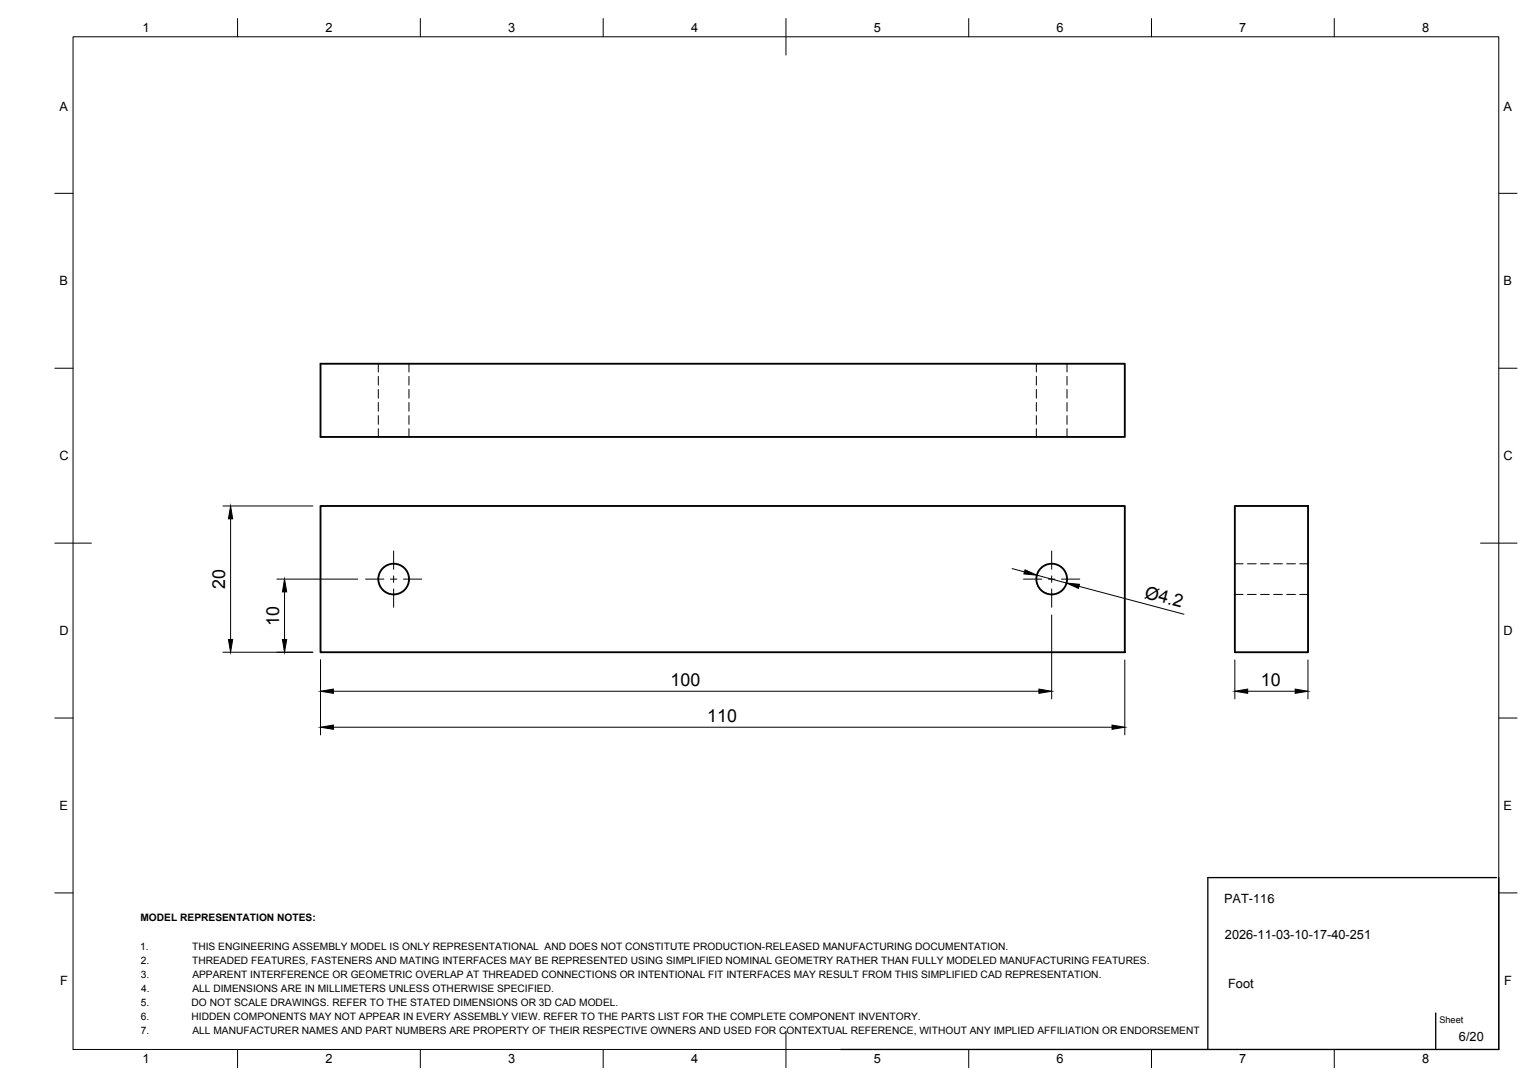
ISO-10303-21;
HEADER;
/* Generated by software containing ST-Developer
 * from STEP Tools, Inc. (www.steptools.com) 
 */

FILE_DESCRIPTION(
/* description */ ('V-block with clamp strap'),
/* implementation_level */ '2;1');

FILE_NAME(
/* name */ 'Foot.step',
/* time_stamp */ '2026-10-27T10:50:53-07:00',
/* author */ (''),
/* organization */ (''),
/* preprocessor_version */ 'ST-DEVELOPER v20.2',
/* originating_system */ 'Autodesk Translation Framework v15.17.0.0',
/* authorisation */ '');

FILE_SCHEMA (('AUTOMOTIVE_DESIGN { 1 0 10303 214 3 1 1 }'));
ENDSEC;

DATA;
#10=MECHANICAL_DESIGN_GEOMETRIC_PRESENTATION_REPRESENTATION('',(#267),#7344);
#225=SHAPE_REPRESENTATION_RELATIONSHIP('SRR','None',#7443,#246);
#246=ADVANCED_BREP_SHAPE_REPRESENTATION('',(#288),#7322);
#267=STYLED_ITEM('',(#7645),#288);
#288=MANIFOLD_SOLID_BREP('Body1',#4149);
#331=FACE_BOUND('',#863,.T.);
#332=FACE_BOUND('',#864,.T.);
#333=FACE_BOUND('',#866,.T.);
#334=FACE_BOUND('',#867,.T.);
#400=CIRCLE('',#4461,0.21);
#401=CIRCLE('',#4462,0.21);
#402=CIRCLE('',#4464,0.21);
#403=CIRCLE('',#4465,0.21);
#517=CYLINDRICAL_SURFACE('',#4460,0.21);
#518=CYLINDRICAL_SURFACE('',#4463,0.21);
#590=FACE_OUTER_BOUND('',#856,.T.);
#591=FACE_OUTER_BOUND('',#857,.T.);
#592=FACE_OUTER_BOUND('',#858,.T.);
#593=FACE_OUTER_BOUND('',#859,.T.);
#594=FACE_OUTER_BOUND('',#860,.T.);
#595=FACE_OUTER_BOUND('',#861,.T.);
#596=FACE_OUTER_BOUND('',#862,.T.);
#597=FACE_OUTER_BOUND('',#865,.T.);
#856=EDGE_LOOP('',(#2840,#2841,#2842,#2843));
#857=EDGE_LOOP('',(#2844,#2845,#2846,#2847));
#858=EDGE_LOOP('',(#2848,#2849,#2850,#2851));
#859=EDGE_LOOP('',(#2852,#2853,#2854,#2855));
#860=EDGE_LOOP('',(#2856,#2857,#2858,#2859));
#861=EDGE_LOOP('',(#2860,#2861,#2862,#2863));
#862=EDGE_LOOP('',(#2864,#2865,#2866,#2867));
#863=EDGE_LOOP('',(#2868));
#864=EDGE_LOOP('',(#2869));
#865=EDGE_LOOP('',(#2870,#2871,#2872,#2873));
#866=EDGE_LOOP('',(#2874));
#867=EDGE_LOOP('',(#2875));
#1161=LINE('',#6242,#1526);
#1162=LINE('',#6248,#1527);
#1163=LINE('',#6253,#1528);
#1164=LINE('',#6255,#1529);
#1165=LINE('',#6257,#1530);
#1166=LINE('',#6258,#1531);
#1167=LINE('',#6261,#1532);
#1168=LINE('',#6263,#1533);
#1169=LINE('',#6264,#1534);
#1170=LINE('',#6267,#1535);
#1171=LINE('',#6269,#1536);
#1172=LINE('',#6270,#1537);
#1173=LINE('',#6272,#1538);
#1174=LINE('',#6273,#1539);
#1526=VECTOR('',#5007,0.21);
#1527=VECTOR('',#5014,0.21);
#1528=VECTOR('',#5019,1.);
#1529=VECTOR('',#5020,1.);
#1530=VECTOR('',#5021,1.);
#1531=VECTOR('',#5022,1.);
#1532=VECTOR('',#5025,1.);
#1533=VECTOR('',#5026,1.);
#1534=VECTOR('',#5027,1.);
#1535=VECTOR('',#5030,1.);
#1536=VECTOR('',#5031,1.);
#1537=VECTOR('',#5032,1.);
#1538=VECTOR('',#5035,1.);
#1539=VECTOR('',#5036,1.);
#1891=VERTEX_POINT('',#6239);
#1892=VERTEX_POINT('',#6241);
#1893=VERTEX_POINT('',#6245);
#1894=VERTEX_POINT('',#6247);
#1895=VERTEX_POINT('',#6251);
#1896=VERTEX_POINT('',#6252);
#1897=VERTEX_POINT('',#6254);
#1898=VERTEX_POINT('',#6256);
#1899=VERTEX_POINT('',#6260);
#1900=VERTEX_POINT('',#6262);
#1901=VERTEX_POINT('',#6266);
#1902=VERTEX_POINT('',#6268);
#2246=EDGE_CURVE('',#1891,#1891,#400,.T.);
#2247=EDGE_CURVE('',#1891,#1892,#1161,.T.);
#2248=EDGE_CURVE('',#1892,#1892,#401,.T.);
#2249=EDGE_CURVE('',#1893,#1893,#402,.T.);
#2250=EDGE_CURVE('',#1893,#1894,#1162,.T.);
#2251=EDGE_CURVE('',#1894,#1894,#403,.T.);
#2252=EDGE_CURVE('',#1895,#1896,#1163,.T.);
#2253=EDGE_CURVE('',#1896,#1897,#1164,.T.);
#2254=EDGE_CURVE('',#1898,#1897,#1165,.T.);
#2255=EDGE_CURVE('',#1895,#1898,#1166,.T.);
#2256=EDGE_CURVE('',#1899,#1895,#1167,.T.);
#2257=EDGE_CURVE('',#1900,#1898,#1168,.T.);
#2258=EDGE_CURVE('',#1899,#1900,#1169,.T.);
#2259=EDGE_CURVE('',#1901,#1899,#1170,.T.);
#2260=EDGE_CURVE('',#1902,#1900,#1171,.T.);
#2261=EDGE_CURVE('',#1901,#1902,#1172,.T.);
#2262=EDGE_CURVE('',#1896,#1901,#1173,.T.);
#2263=EDGE_CURVE('',#1897,#1902,#1174,.T.);
#2840=ORIENTED_EDGE('',*,*,#2246,.F.);
#2841=ORIENTED_EDGE('',*,*,#2247,.T.);
#2842=ORIENTED_EDGE('',*,*,#2248,.F.);
#2843=ORIENTED_EDGE('',*,*,#2247,.F.);
#2844=ORIENTED_EDGE('',*,*,#2249,.F.);
#2845=ORIENTED_EDGE('',*,*,#2250,.T.);
#2846=ORIENTED_EDGE('',*,*,#2251,.F.);
#2847=ORIENTED_EDGE('',*,*,#2250,.F.);
#2848=ORIENTED_EDGE('',*,*,#2252,.T.);
#2849=ORIENTED_EDGE('',*,*,#2253,.T.);
#2850=ORIENTED_EDGE('',*,*,#2254,.F.);
#2851=ORIENTED_EDGE('',*,*,#2255,.F.);
#2852=ORIENTED_EDGE('',*,*,#2256,.T.);
#2853=ORIENTED_EDGE('',*,*,#2255,.T.);
#2854=ORIENTED_EDGE('',*,*,#2257,.F.);
#2855=ORIENTED_EDGE('',*,*,#2258,.F.);
#2856=ORIENTED_EDGE('',*,*,#2259,.T.);
#2857=ORIENTED_EDGE('',*,*,#2258,.T.);
#2858=ORIENTED_EDGE('',*,*,#2260,.F.);
#2859=ORIENTED_EDGE('',*,*,#2261,.F.);
#2860=ORIENTED_EDGE('',*,*,#2262,.T.);
#2861=ORIENTED_EDGE('',*,*,#2261,.T.);
#2862=ORIENTED_EDGE('',*,*,#2263,.F.);
#2863=ORIENTED_EDGE('',*,*,#2253,.F.);
#2864=ORIENTED_EDGE('',*,*,#2263,.T.);
#2865=ORIENTED_EDGE('',*,*,#2260,.T.);
#2866=ORIENTED_EDGE('',*,*,#2257,.T.);
#2867=ORIENTED_EDGE('',*,*,#2254,.T.);
#2868=ORIENTED_EDGE('',*,*,#2248,.T.);
#2869=ORIENTED_EDGE('',*,*,#2251,.T.);
#2870=ORIENTED_EDGE('',*,*,#2262,.F.);
#2871=ORIENTED_EDGE('',*,*,#2252,.F.);
#2872=ORIENTED_EDGE('',*,*,#2256,.F.);
#2873=ORIENTED_EDGE('',*,*,#2259,.F.);
#2874=ORIENTED_EDGE('',*,*,#2246,.T.);
#2875=ORIENTED_EDGE('',*,*,#2249,.T.);
#3756=PLANE('',#4466);
#3757=PLANE('',#4467);
#3758=PLANE('',#4468);
#3759=PLANE('',#4469);
#3760=PLANE('',#4470);
#3761=PLANE('',#4471);
#3936=ADVANCED_FACE('',(#590),#517,.F.);
#3937=ADVANCED_FACE('',(#591),#518,.F.);
#3938=ADVANCED_FACE('',(#592),#3756,.T.);
#3939=ADVANCED_FACE('',(#593),#3757,.T.);
#3940=ADVANCED_FACE('',(#594),#3758,.T.);
#3941=ADVANCED_FACE('',(#595),#3759,.T.);
#3942=ADVANCED_FACE('',(#596,#331,#332),#3760,.T.);
#3943=ADVANCED_FACE('',(#597,#333,#334),#3761,.F.);
#4149=CLOSED_SHELL('',(#3936,#3937,#3938,#3939,#3940,#3941,#3942,#3943));
#4459=AXIS2_PLACEMENT_3D('',#6237,#5001,#5002);
#4460=AXIS2_PLACEMENT_3D('',#6238,#5003,#5004);
#4461=AXIS2_PLACEMENT_3D('',#6240,#5005,#5006);
#4462=AXIS2_PLACEMENT_3D('',#6243,#5008,#5009);
#4463=AXIS2_PLACEMENT_3D('',#6244,#5010,#5011);
#4464=AXIS2_PLACEMENT_3D('',#6246,#5012,#5013);
#4465=AXIS2_PLACEMENT_3D('',#6249,#5015,#5016);
#4466=AXIS2_PLACEMENT_3D('',#6250,#5017,#5018);
#4467=AXIS2_PLACEMENT_3D('',#6259,#5023,#5024);
#4468=AXIS2_PLACEMENT_3D('',#6265,#5028,#5029);
#4469=AXIS2_PLACEMENT_3D('',#6271,#5033,#5034);
#4470=AXIS2_PLACEMENT_3D('',#6274,#5037,#5038);
#4471=AXIS2_PLACEMENT_3D('',#6275,#5039,#5040);
#5001=DIRECTION('axis',(0.,0.,1.));
#5002=DIRECTION('refdir',(1.,0.,0.));
#5003=DIRECTION('center_axis',(0.,0.,1.));
#5004=DIRECTION('ref_axis',(1.,0.,0.));
#5005=DIRECTION('center_axis',(0.,0.,1.));
#5006=DIRECTION('ref_axis',(1.,0.,0.));
#5007=DIRECTION('',(0.,0.,1.));
#5008=DIRECTION('center_axis',(0.,0.,-1.));
#5009=DIRECTION('ref_axis',(1.,0.,0.));
#5010=DIRECTION('center_axis',(0.,0.,1.));
#5011=DIRECTION('ref_axis',(1.,0.,0.));
#5012=DIRECTION('center_axis',(0.,0.,1.));
#5013=DIRECTION('ref_axis',(1.,0.,0.));
#5014=DIRECTION('',(0.,0.,1.));
#5015=DIRECTION('center_axis',(0.,0.,-1.));
#5016=DIRECTION('ref_axis',(1.,0.,0.));
#5017=DIRECTION('center_axis',(0.,1.,0.));
#5018=DIRECTION('ref_axis',(-1.,0.,0.));
#5019=DIRECTION('',(-1.,0.,0.));
#5020=DIRECTION('',(0.,0.,1.));
#5021=DIRECTION('',(-1.,0.,0.));
#5022=DIRECTION('',(0.,0.,1.));
#5023=DIRECTION('center_axis',(1.,0.,0.));
#5024=DIRECTION('ref_axis',(0.,1.,0.));
#5025=DIRECTION('',(0.,1.,0.));
#5026=DIRECTION('',(0.,1.,0.));
#5027=DIRECTION('',(0.,0.,1.));
#5028=DIRECTION('center_axis',(0.,-1.,0.));
#5029=DIRECTION('ref_axis',(1.,0.,0.));
#5030=DIRECTION('',(1.,0.,0.));
#5031=DIRECTION('',(1.,0.,0.));
#5032=DIRECTION('',(0.,0.,1.));
#5033=DIRECTION('center_axis',(-1.,0.,0.));
#5034=DIRECTION('ref_axis',(0.,-1.,0.));
#5035=DIRECTION('',(0.,-1.,0.));
#5036=DIRECTION('',(0.,-1.,0.));
#5037=DIRECTION('center_axis',(0.,0.,1.));
#5038=DIRECTION('ref_axis',(1.,0.,0.));
#5039=DIRECTION('center_axis',(0.,0.,1.));
#5040=DIRECTION('ref_axis',(1.,0.,0.));
#6237=CARTESIAN_POINT('',(0.,0.,0.));
#6238=CARTESIAN_POINT('Origin',(3.,-4.5,-1.1));
#6239=CARTESIAN_POINT('',(2.79,-4.5,-1.));
#6240=CARTESIAN_POINT('Origin',(3.,-4.5,-1.));
#6241=CARTESIAN_POINT('',(2.79,-4.5,0.));
#6242=CARTESIAN_POINT('',(2.79,-4.5,-1.1));
#6243=CARTESIAN_POINT('Origin',(3.,-4.5,0.));
#6244=CARTESIAN_POINT('Origin',(3.,4.5,-1.1));
#6245=CARTESIAN_POINT('',(2.79,4.5,-1.));
#6246=CARTESIAN_POINT('Origin',(3.,4.5,-1.));
#6247=CARTESIAN_POINT('',(2.79,4.5,0.));
#6248=CARTESIAN_POINT('',(2.79,4.5,-1.1));
#6249=CARTESIAN_POINT('Origin',(3.,4.5,0.));
#6250=CARTESIAN_POINT('Origin',(4.,5.5,-1.));
#6251=CARTESIAN_POINT('',(4.,5.5,-1.));
#6252=CARTESIAN_POINT('',(2.,5.5,-1.));
#6253=CARTESIAN_POINT('',(4.,5.5,-1.));
#6254=CARTESIAN_POINT('',(2.,5.5,0.));
#6255=CARTESIAN_POINT('',(2.,5.5,-1.));
#6256=CARTESIAN_POINT('',(4.,5.5,0.));
#6257=CARTESIAN_POINT('',(4.,5.5,0.));
#6258=CARTESIAN_POINT('',(4.,5.5,-1.));
#6259=CARTESIAN_POINT('Origin',(4.,-5.5,-1.));
#6260=CARTESIAN_POINT('',(4.,-5.5,-1.));
#6261=CARTESIAN_POINT('',(4.,-5.5,-1.));
#6262=CARTESIAN_POINT('',(4.,-5.5,0.));
#6263=CARTESIAN_POINT('',(4.,-5.5,0.));
#6264=CARTESIAN_POINT('',(4.,-5.5,-1.));
#6265=CARTESIAN_POINT('Origin',(2.,-5.5,-1.));
#6266=CARTESIAN_POINT('',(2.,-5.5,-1.));
#6267=CARTESIAN_POINT('',(2.,-5.5,-1.));
#6268=CARTESIAN_POINT('',(2.,-5.5,0.));
#6269=CARTESIAN_POINT('',(2.,-5.5,0.));
#6270=CARTESIAN_POINT('',(2.,-5.5,-1.));
#6271=CARTESIAN_POINT('Origin',(2.,5.5,-1.));
#6272=CARTESIAN_POINT('',(2.,5.5,-1.));
#6273=CARTESIAN_POINT('',(2.,5.5,0.));
#6274=CARTESIAN_POINT('Origin',(3.,0.,0.));
#6275=CARTESIAN_POINT('Origin',(3.,0.,-1.));
#7296=UNCERTAINTY_MEASURE_WITH_UNIT(LENGTH_MEASURE(0.001),#7345,
'DISTANCE_ACCURACY_VALUE',
'Maximum model space distance between geometric entities at asserted c
onnectivities');
#7318=UNCERTAINTY_MEASURE_WITH_UNIT(LENGTH_MEASURE(0.001),#7345,
'DISTANCE_ACCURACY_VALUE',
'Maximum model space distance between geometric entities at asserted c
onnectivities');
#7322=(
GEOMETRIC_REPRESENTATION_CONTEXT(3)
GLOBAL_UNCERTAINTY_ASSIGNED_CONTEXT((#7296))
GLOBAL_UNIT_ASSIGNED_CONTEXT((#7345,#7347,#7348))
REPRESENTATION_CONTEXT('','3D')
);
#7344=(
GEOMETRIC_REPRESENTATION_CONTEXT(3)
GLOBAL_UNCERTAINTY_ASSIGNED_CONTEXT((#7318))
GLOBAL_UNIT_ASSIGNED_CONTEXT((#7345,#7347,#7348))
REPRESENTATION_CONTEXT('','3D')
);
#7345=(
LENGTH_UNIT()
NAMED_UNIT(*)
SI_UNIT(.CENTI.,.METRE.)
);
#7347=(
NAMED_UNIT(*)
PLANE_ANGLE_UNIT()
SI_UNIT($,.RADIAN.)
);
#7348=(
NAMED_UNIT(*)
SI_UNIT($,.STERADIAN.)
SOLID_ANGLE_UNIT()
);
#7352=SHAPE_DEFINITION_REPRESENTATION(#7377,#7443);
#7377=PRODUCT_DEFINITION_SHAPE('',$,#7469);
#7443=SHAPE_REPRESENTATION('',(#4459),#7322);
#7465=PRODUCT_DEFINITION_CONTEXT('part definition',#7542,'design');
#7469=PRODUCT_DEFINITION('Foot','Foot',#7494,#7465);
#7494=PRODUCT_DEFINITION_FORMATION('',$,#7547);
#7542=APPLICATION_CONTEXT(
'Core Data for Automotive Mechanical Design Process');
#7543=PRODUCT_CONTEXT('part definition',#7542,'mechanical');
#7547=PRODUCT('Foot','Foot','Foot',(#7543));
#7639=COLOUR_RGB('Off White',0.89,0.88,0.83);
#7640=FILL_AREA_STYLE_COLOUR('',#7639);
#7641=FILL_AREA_STYLE('',(#7640));
#7642=SURFACE_STYLE_FILL_AREA(#7641);
#7643=SURFACE_SIDE_STYLE('',(#7642));
#7644=SURFACE_STYLE_USAGE(.BOTH.,#7643);
#7645=PRESENTATION_STYLE_ASSIGNMENT((#7644));
ENDSEC;
END-ISO-10303-21;
